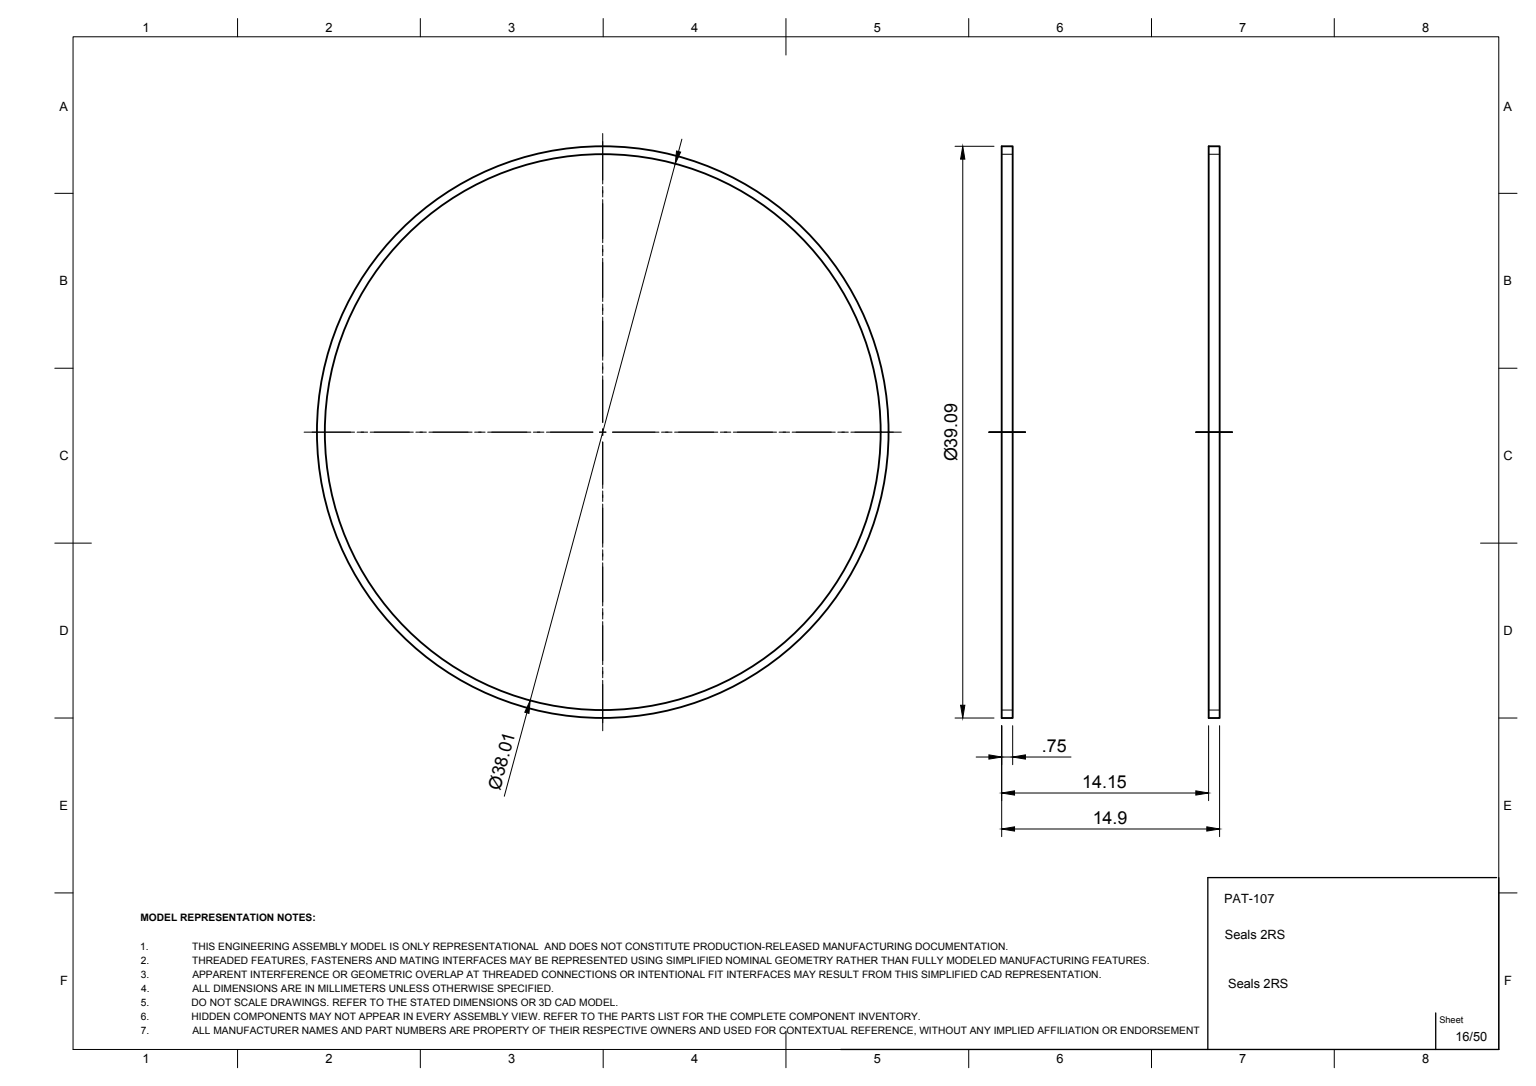
ISO-10303-21;
HEADER;
/* Generated by software containing ST-Developer
 * from STEP Tools, Inc. (www.steptools.com) 
 */

FILE_DESCRIPTION(
/* description */ ('Turntable on roller ring'),
/* implementation_level */ '2;1');

FILE_NAME(
/* name */ 'Seals 2RS.step',
/* time_stamp */ '2026-10-28T03:23:59-07:00',
/* author */ (''),
/* organization */ (''),
/* preprocessor_version */ 'ST-DEVELOPER v20.2',
/* originating_system */ 'Autodesk Translation Framework v15.17.0.0',
/* authorisation */ '');

FILE_SCHEMA (('AUTOMOTIVE_DESIGN { 1 0 10303 214 3 1 1 }'));
ENDSEC;

DATA;
#10=MECHANICAL_DESIGN_GEOMETRIC_PRESENTATION_REPRESENTATION('',(#633,#634),#16281);
#515=SHAPE_REPRESENTATION_RELATIONSHIP('SRR','None',#16530,#570);
#570=ADVANCED_BREP_SHAPE_REPRESENTATION('',(#704,#705),#16224);
#633=STYLED_ITEM('',(#16932),#704);
#634=STYLED_ITEM('',(#16932),#705);
#704=MANIFOLD_SOLID_BREP('Body1',#8375);
#705=MANIFOLD_SOLID_BREP('Body2',#8376);
#829=FACE_BOUND('',#1956,.T.);
#830=FACE_BOUND('',#1959,.T.);
#831=FACE_BOUND('',#1962,.T.);
#832=FACE_BOUND('',#1965,.T.);
#1035=PLANE('',#9353);
#1036=PLANE('',#9358);
#1037=PLANE('',#9361);
#1038=PLANE('',#9366);
#1378=FACE_OUTER_BOUND('',#1955,.T.);
#1379=FACE_OUTER_BOUND('',#1957,.T.);
#1380=FACE_OUTER_BOUND('',#1958,.T.);
#1381=FACE_OUTER_BOUND('',#1960,.T.);
#1382=FACE_OUTER_BOUND('',#1961,.T.);
#1383=FACE_OUTER_BOUND('',#1963,.T.);
#1384=FACE_OUTER_BOUND('',#1964,.T.);
#1385=FACE_OUTER_BOUND('',#1966,.T.);
#1955=EDGE_LOOP('',(#6221));
#1956=EDGE_LOOP('',(#6222));
#1957=EDGE_LOOP('',(#6223,#6224,#6225,#6226));
#1958=EDGE_LOOP('',(#6227));
#1959=EDGE_LOOP('',(#6228));
#1960=EDGE_LOOP('',(#6229,#6230,#6231,#6232));
#1961=EDGE_LOOP('',(#6233));
#1962=EDGE_LOOP('',(#6234));
#1963=EDGE_LOOP('',(#6235,#6236,#6237,#6238));
#1964=EDGE_LOOP('',(#6239));
#1965=EDGE_LOOP('',(#6240));
#1966=EDGE_LOOP('',(#6241,#6242,#6243,#6244));
#2590=LINE('',#14013,#3073);
#2591=LINE('',#14018,#3074);
#2592=LINE('',#14027,#3075);
#2593=LINE('',#14032,#3076);
#3073=VECTOR('',#10933,1.95469);
#3074=VECTOR('',#10940,1.90031);
#3075=VECTOR('',#10951,1.95469);
#3076=VECTOR('',#10958,1.90031);
#3632=CIRCLE('',#9354,1.95469);
#3633=CIRCLE('',#9355,1.90031);
#3634=CIRCLE('',#9357,1.95469);
#3635=CIRCLE('',#9359,1.90031);
#3636=CIRCLE('',#9362,1.95469);
#3637=CIRCLE('',#9363,1.90031);
#3638=CIRCLE('',#9365,1.95469);
#3639=CIRCLE('',#9367,1.90031);
#4145=VERTEX_POINT('',#14006);
#4146=VERTEX_POINT('',#14008);
#4147=VERTEX_POINT('',#14011);
#4148=VERTEX_POINT('',#14015);
#4149=VERTEX_POINT('',#14020);
#4150=VERTEX_POINT('',#14022);
#4151=VERTEX_POINT('',#14025);
#4152=VERTEX_POINT('',#14029);
#4921=EDGE_CURVE('',#4145,#4145,#3632,.T.);
#4922=EDGE_CURVE('',#4146,#4146,#3633,.T.);
#4923=EDGE_CURVE('',#4147,#4147,#3634,.T.);
#4924=EDGE_CURVE('',#4147,#4145,#2590,.T.);
#4925=EDGE_CURVE('',#4148,#4148,#3635,.T.);
#4926=EDGE_CURVE('',#4148,#4146,#2591,.T.);
#4927=EDGE_CURVE('',#4149,#4149,#3636,.T.);
#4928=EDGE_CURVE('',#4150,#4150,#3637,.T.);
#4929=EDGE_CURVE('',#4151,#4151,#3638,.T.);
#4930=EDGE_CURVE('',#4151,#4149,#2592,.T.);
#4931=EDGE_CURVE('',#4152,#4152,#3639,.T.);
#4932=EDGE_CURVE('',#4152,#4150,#2593,.T.);
#6221=ORIENTED_EDGE('',*,*,#4921,.F.);
#6222=ORIENTED_EDGE('',*,*,#4922,.T.);
#6223=ORIENTED_EDGE('',*,*,#4923,.F.);
#6224=ORIENTED_EDGE('',*,*,#4924,.T.);
#6225=ORIENTED_EDGE('',*,*,#4921,.T.);
#6226=ORIENTED_EDGE('',*,*,#4924,.F.);
#6227=ORIENTED_EDGE('',*,*,#4923,.T.);
#6228=ORIENTED_EDGE('',*,*,#4925,.F.);
#6229=ORIENTED_EDGE('',*,*,#4925,.T.);
#6230=ORIENTED_EDGE('',*,*,#4926,.T.);
#6231=ORIENTED_EDGE('',*,*,#4922,.F.);
#6232=ORIENTED_EDGE('',*,*,#4926,.F.);
#6233=ORIENTED_EDGE('',*,*,#4927,.F.);
#6234=ORIENTED_EDGE('',*,*,#4928,.T.);
#6235=ORIENTED_EDGE('',*,*,#4929,.F.);
#6236=ORIENTED_EDGE('',*,*,#4930,.T.);
#6237=ORIENTED_EDGE('',*,*,#4927,.T.);
#6238=ORIENTED_EDGE('',*,*,#4930,.F.);
#6239=ORIENTED_EDGE('',*,*,#4929,.T.);
#6240=ORIENTED_EDGE('',*,*,#4931,.F.);
#6241=ORIENTED_EDGE('',*,*,#4931,.T.);
#6242=ORIENTED_EDGE('',*,*,#4932,.T.);
#6243=ORIENTED_EDGE('',*,*,#4928,.F.);
#6244=ORIENTED_EDGE('',*,*,#4932,.F.);
#7725=CYLINDRICAL_SURFACE('',#9356,1.95469);
#7726=CYLINDRICAL_SURFACE('',#9360,1.90031);
#7727=CYLINDRICAL_SURFACE('',#9364,1.95469);
#7728=CYLINDRICAL_SURFACE('',#9368,1.90031);
#7981=ADVANCED_FACE('',(#1378,#829),#1035,.T.);
#7982=ADVANCED_FACE('',(#1379),#7725,.T.);
#7983=ADVANCED_FACE('',(#1380,#830),#1036,.T.);
#7984=ADVANCED_FACE('',(#1381),#7726,.F.);
#7985=ADVANCED_FACE('',(#1382,#831),#1037,.T.);
#7986=ADVANCED_FACE('',(#1383),#7727,.T.);
#7987=ADVANCED_FACE('',(#1384,#832),#1038,.T.);
#7988=ADVANCED_FACE('',(#1385),#7728,.F.);
#8375=CLOSED_SHELL('',(#7981,#7982,#7983,#7984));
#8376=CLOSED_SHELL('',(#7985,#7986,#7987,#7988));
#9352=AXIS2_PLACEMENT_3D('',#14004,#10921,#10922);
#9353=AXIS2_PLACEMENT_3D('',#14005,#10923,#10924);
#9354=AXIS2_PLACEMENT_3D('',#14007,#10925,#10926);
#9355=AXIS2_PLACEMENT_3D('',#14009,#10927,#10928);
#9356=AXIS2_PLACEMENT_3D('',#14010,#10929,#10930);
#9357=AXIS2_PLACEMENT_3D('',#14012,#10931,#10932);
#9358=AXIS2_PLACEMENT_3D('',#14014,#10934,#10935);
#9359=AXIS2_PLACEMENT_3D('',#14016,#10936,#10937);
#9360=AXIS2_PLACEMENT_3D('',#14017,#10938,#10939);
#9361=AXIS2_PLACEMENT_3D('',#14019,#10941,#10942);
#9362=AXIS2_PLACEMENT_3D('',#14021,#10943,#10944);
#9363=AXIS2_PLACEMENT_3D('',#14023,#10945,#10946);
#9364=AXIS2_PLACEMENT_3D('',#14024,#10947,#10948);
#9365=AXIS2_PLACEMENT_3D('',#14026,#10949,#10950);
#9366=AXIS2_PLACEMENT_3D('',#14028,#10952,#10953);
#9367=AXIS2_PLACEMENT_3D('',#14030,#10954,#10955);
#9368=AXIS2_PLACEMENT_3D('',#14031,#10956,#10957);
#10921=DIRECTION('axis',(0.,0.,1.));
#10922=DIRECTION('refdir',(1.,0.,0.));
#10923=DIRECTION('center_axis',(0.,1.,0.));
#10924=DIRECTION('ref_axis',(0.,0.,1.));
#10925=DIRECTION('center_axis',(0.,-1.,0.));
#10926=DIRECTION('ref_axis',(1.,0.,0.));
#10927=DIRECTION('center_axis',(0.,-1.,0.));
#10928=DIRECTION('ref_axis',(1.,0.,0.));
#10929=DIRECTION('center_axis',(0.,-1.,0.));
#10930=DIRECTION('ref_axis',(1.,0.,0.));
#10931=DIRECTION('center_axis',(0.,-1.,0.));
#10932=DIRECTION('ref_axis',(1.,0.,0.));
#10933=DIRECTION('',(0.,1.,0.));
#10934=DIRECTION('center_axis',(0.,-1.,0.));
#10935=DIRECTION('ref_axis',(0.,0.,-1.));
#10936=DIRECTION('center_axis',(0.,-1.,0.));
#10937=DIRECTION('ref_axis',(1.,0.,0.));
#10938=DIRECTION('center_axis',(0.,-1.,0.));
#10939=DIRECTION('ref_axis',(1.,0.,0.));
#10940=DIRECTION('',(0.,1.,0.));
#10941=DIRECTION('center_axis',(0.,1.,0.));
#10942=DIRECTION('ref_axis',(0.,0.,1.));
#10943=DIRECTION('center_axis',(0.,-1.,0.));
#10944=DIRECTION('ref_axis',(1.,0.,0.));
#10945=DIRECTION('center_axis',(0.,-1.,0.));
#10946=DIRECTION('ref_axis',(1.,0.,0.));
#10947=DIRECTION('center_axis',(0.,-1.,0.));
#10948=DIRECTION('ref_axis',(1.,0.,0.));
#10949=DIRECTION('center_axis',(0.,-1.,0.));
#10950=DIRECTION('ref_axis',(1.,0.,0.));
#10951=DIRECTION('',(0.,1.,0.));
#10952=DIRECTION('center_axis',(0.,-1.,0.));
#10953=DIRECTION('ref_axis',(0.,0.,-1.));
#10954=DIRECTION('center_axis',(0.,-1.,0.));
#10955=DIRECTION('ref_axis',(1.,0.,0.));
#10956=DIRECTION('center_axis',(0.,-1.,0.));
#10957=DIRECTION('ref_axis',(1.,0.,0.));
#10958=DIRECTION('',(0.,1.,0.));
#14004=CARTESIAN_POINT('',(0.,0.,0.));
#14005=CARTESIAN_POINT('Origin',(1.95469,0.745,0.));
#14006=CARTESIAN_POINT('',(-1.95469,0.745,-2.39380485182534E-16));
#14007=CARTESIAN_POINT('Origin',(0.,0.745,0.));
#14008=CARTESIAN_POINT('',(-1.90031,0.745,-2.32720855888771E-16));
#14009=CARTESIAN_POINT('Origin',(0.,0.745,0.));
#14010=CARTESIAN_POINT('Origin',(0.,0.7075,0.));
#14011=CARTESIAN_POINT('',(-1.95469,0.67,-2.39380485182534E-16));
#14012=CARTESIAN_POINT('Origin',(0.,0.67,0.));
#14013=CARTESIAN_POINT('',(-1.95469,0.7075,-2.39380485182534E-16));
#14014=CARTESIAN_POINT('Origin',(1.90031,0.67,0.));
#14015=CARTESIAN_POINT('',(-1.90031,0.67,-2.32720855888771E-16));
#14016=CARTESIAN_POINT('Origin',(0.,0.67,0.));
#14017=CARTESIAN_POINT('Origin',(0.,0.7075,0.));
#14018=CARTESIAN_POINT('',(-1.90031,0.7075,-2.32720855888771E-16));
#14019=CARTESIAN_POINT('Origin',(1.95469,-0.67,0.));
#14020=CARTESIAN_POINT('',(-1.95469,-0.67,-2.39380485182534E-16));
#14021=CARTESIAN_POINT('Origin',(0.,-0.67,0.));
#14022=CARTESIAN_POINT('',(-1.90031,-0.67,-2.32720855888771E-16));
#14023=CARTESIAN_POINT('Origin',(0.,-0.67,0.));
#14024=CARTESIAN_POINT('Origin',(0.,-0.7075,0.));
#14025=CARTESIAN_POINT('',(-1.95469,-0.745,-2.39380485182534E-16));
#14026=CARTESIAN_POINT('Origin',(0.,-0.745,0.));
#14027=CARTESIAN_POINT('',(-1.95469,-0.7075,-2.39380485182534E-16));
#14028=CARTESIAN_POINT('Origin',(1.90031,-0.745,0.));
#14029=CARTESIAN_POINT('',(-1.90031,-0.745,-2.32720855888771E-16));
#14030=CARTESIAN_POINT('Origin',(0.,-0.745,0.));
#14031=CARTESIAN_POINT('Origin',(0.,-0.7075,0.));
#14032=CARTESIAN_POINT('',(-1.90031,-0.7075,-2.32720855888771E-16));
#16155=UNCERTAINTY_MEASURE_WITH_UNIT(LENGTH_MEASURE(0.001),#16282,
'DISTANCE_ACCURACY_VALUE',
'Maximum model space distance between geometric entities at asserted c
onnectivities');
#16212=UNCERTAINTY_MEASURE_WITH_UNIT(LENGTH_MEASURE(0.001),#16282,
'DISTANCE_ACCURACY_VALUE',
'Maximum model space distance between geometric entities at asserted c
onnectivities');
#16224=(
GEOMETRIC_REPRESENTATION_CONTEXT(3)
GLOBAL_UNCERTAINTY_ASSIGNED_CONTEXT((#16155))
GLOBAL_UNIT_ASSIGNED_CONTEXT((#16282,#16284,#16285))
REPRESENTATION_CONTEXT('','3D')
);
#16281=(
GEOMETRIC_REPRESENTATION_CONTEXT(3)
GLOBAL_UNCERTAINTY_ASSIGNED_CONTEXT((#16212))
GLOBAL_UNIT_ASSIGNED_CONTEXT((#16282,#16284,#16285))
REPRESENTATION_CONTEXT('','3D')
);
#16282=(
LENGTH_UNIT()
NAMED_UNIT(*)
SI_UNIT(.CENTI.,.METRE.)
);
#16284=(
NAMED_UNIT(*)
PLANE_ANGLE_UNIT()
SI_UNIT($,.RADIAN.)
);
#16285=(
NAMED_UNIT(*)
SI_UNIT($,.STERADIAN.)
SOLID_ANGLE_UNIT()
);
#16297=SHAPE_DEFINITION_REPRESENTATION(#16365,#16530);
#16365=PRODUCT_DEFINITION_SHAPE('',$,#16599);
#16530=SHAPE_REPRESENTATION('',(#9352),#16224);
#16587=PRODUCT_DEFINITION_CONTEXT('part definition',#16793,'design');
#16599=PRODUCT_DEFINITION('Seals 2RS','Seals 2RS',#16667,#16587);
#16667=PRODUCT_DEFINITION_FORMATION('',$,#16806);
#16793=APPLICATION_CONTEXT(
'Core Data for Automotive Mechanical Design Process');
#16794=PRODUCT_CONTEXT('part definition',#16793,'mechanical');
#16806=PRODUCT('Seals 2RS','Seals 2RS','Seals 2RS',(#16794));
#16926=COLOUR_RGB('Grey',0.48,0.52,0.57);
#16927=FILL_AREA_STYLE_COLOUR('',#16926);
#16928=FILL_AREA_STYLE('',(#16927));
#16929=SURFACE_STYLE_FILL_AREA(#16928);
#16930=SURFACE_SIDE_STYLE('',(#16929));
#16931=SURFACE_STYLE_USAGE(.BOTH.,#16930);
#16932=PRESENTATION_STYLE_ASSIGNMENT((#16931));
ENDSEC;
END-ISO-10303-21;
